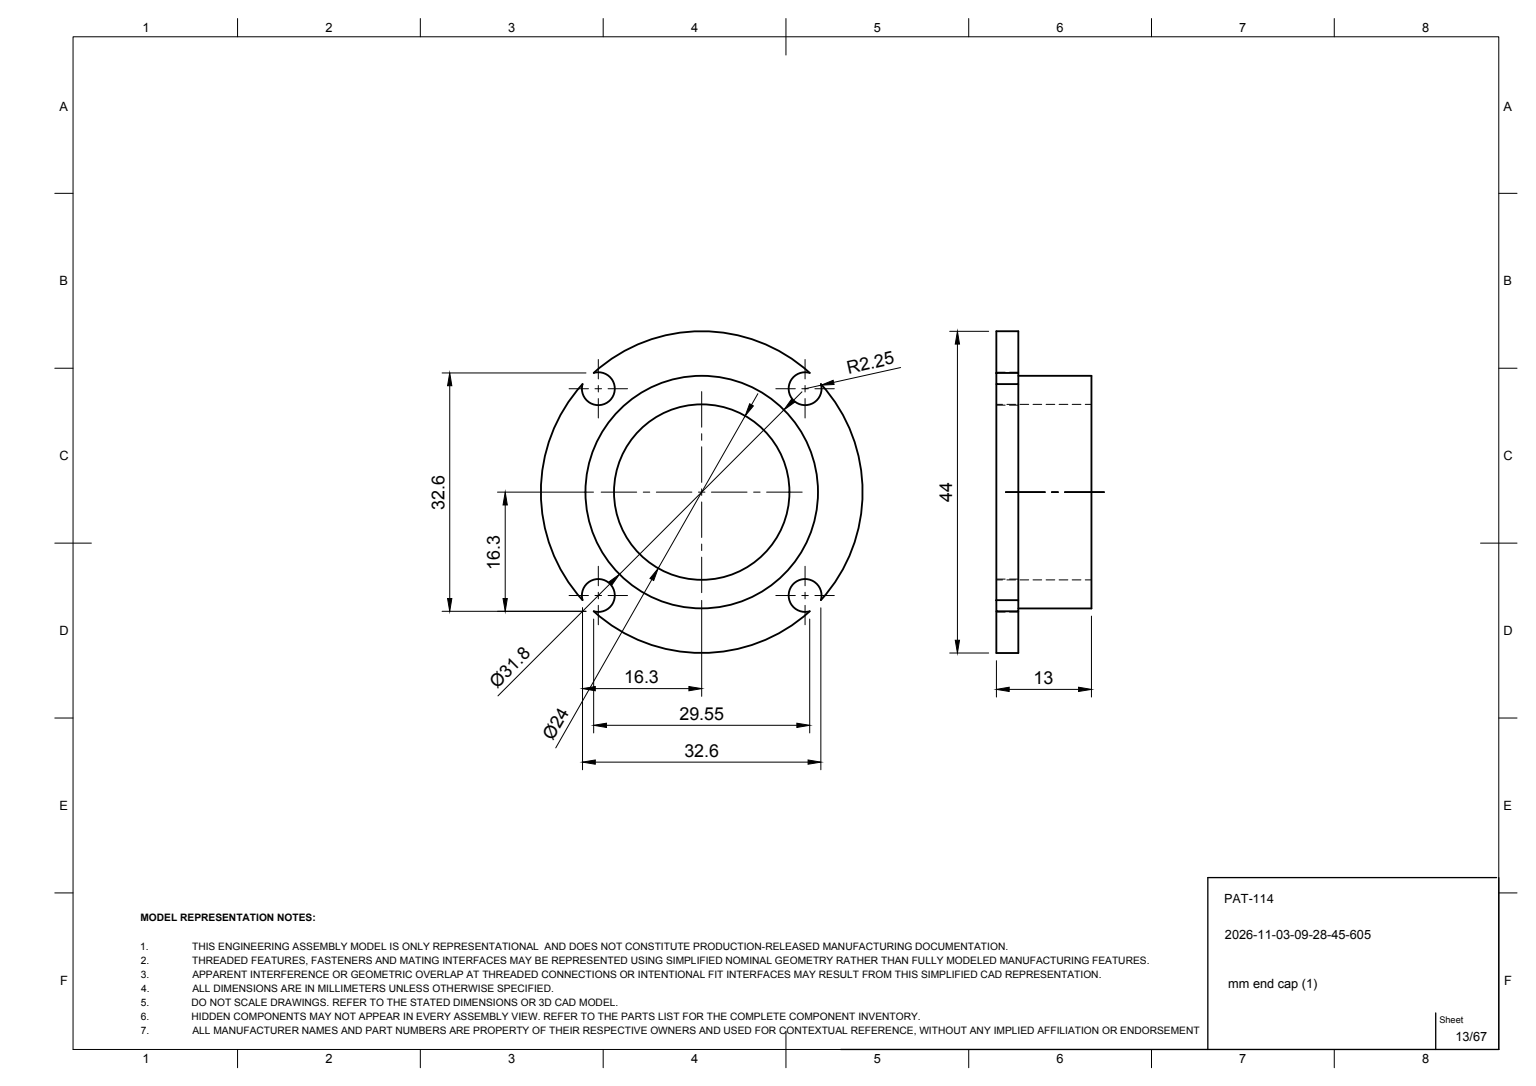
ISO-10303-21;
HEADER;
/* Generated by software containing ST-Developer
 * from STEP Tools, Inc. (www.steptools.com) 
 */

FILE_DESCRIPTION(
/* description */ ('Two-stage gear reducer in split housing'),
/* implementation_level */ '2;1');

FILE_NAME(
/* name */ 'mm end cap (1).step',
/* time_stamp */ '2026-10-28T03:22:31-07:00',
/* author */ (''),
/* organization */ (''),
/* preprocessor_version */ 'ST-DEVELOPER v20.2',
/* originating_system */ 'Autodesk Translation Framework v15.17.0.0',
/* authorisation */ '');

FILE_SCHEMA (('AUTOMOTIVE_DESIGN { 1 0 10303 214 3 1 1 }'));
ENDSEC;

DATA;
#10=MECHANICAL_DESIGN_GEOMETRIC_PRESENTATION_REPRESENTATION('',(#1242),#73366);
#1130=SHAPE_REPRESENTATION_RELATIONSHIP('SRR','None',#73617,#1186);
#1186=ADVANCED_BREP_SHAPE_REPRESENTATION('',(#1313),#73313);
#1242=STYLED_ITEM('',(#74002),#1313);
#1313=MANIFOLD_SOLID_BREP('Body1',#16130);
#1463=FACE_BOUND('',#3216,.T.);
#1464=FACE_BOUND('',#3223,.T.);
#1465=FACE_BOUND('',#3226,.T.);
#1711=PLANE('',#17238);
#1712=PLANE('',#17254);
#1713=PLANE('',#17258);
#2209=FACE_OUTER_BOUND('',#3211,.T.);
#2210=FACE_OUTER_BOUND('',#3212,.T.);
#2211=FACE_OUTER_BOUND('',#3213,.T.);
#2212=FACE_OUTER_BOUND('',#3214,.T.);
#2213=FACE_OUTER_BOUND('',#3215,.T.);
#2214=FACE_OUTER_BOUND('',#3217,.T.);
#2215=FACE_OUTER_BOUND('',#3218,.T.);
#2216=FACE_OUTER_BOUND('',#3219,.T.);
#2217=FACE_OUTER_BOUND('',#3220,.T.);
#2218=FACE_OUTER_BOUND('',#3221,.T.);
#2219=FACE_OUTER_BOUND('',#3222,.T.);
#2220=FACE_OUTER_BOUND('',#3224,.T.);
#2221=FACE_OUTER_BOUND('',#3225,.T.);
#3211=EDGE_LOOP('',(#11431,#11432,#11433,#11434));
#3212=EDGE_LOOP('',(#11435,#11436,#11437,#11438));
#3213=EDGE_LOOP('',(#11439,#11440,#11441,#11442));
#3214=EDGE_LOOP('',(#11443,#11444,#11445,#11446));
#3215=EDGE_LOOP('',(#11447,#11448,#11449,#11450,#11451,#11452,#11453,#11454));
#3216=EDGE_LOOP('',(#11455));
#3217=EDGE_LOOP('',(#11456,#11457,#11458,#11459));
#3218=EDGE_LOOP('',(#11460,#11461,#11462,#11463));
#3219=EDGE_LOOP('',(#11464,#11465,#11466,#11467));
#3220=EDGE_LOOP('',(#11468,#11469,#11470,#11471));
#3221=EDGE_LOOP('',(#11472,#11473,#11474,#11475));
#3222=EDGE_LOOP('',(#11476));
#3223=EDGE_LOOP('',(#11477));
#3224=EDGE_LOOP('',(#11478,#11479,#11480,#11481));
#3225=EDGE_LOOP('',(#11482,#11483,#11484,#11485,#11486,#11487,#11488,#11489));
#3226=EDGE_LOOP('',(#11490));
#4322=LINE('',#23765,#5346);
#4323=LINE('',#23769,#5347);
#4324=LINE('',#23774,#5348);
#4325=LINE('',#23778,#5349);
#4326=LINE('',#23783,#5350);
#4327=LINE('',#23787,#5351);
#4328=LINE('',#23792,#5352);
#4329=LINE('',#23796,#5353);
#4330=LINE('',#23815,#5354);
#4331=LINE('',#23823,#5355);
#5346=VECTOR('',#19554,1.);
#5347=VECTOR('',#19557,1.);
#5348=VECTOR('',#19562,1.);
#5349=VECTOR('',#19565,1.);
#5350=VECTOR('',#19570,1.);
#5351=VECTOR('',#19573,1.);
#5352=VECTOR('',#19578,1.);
#5353=VECTOR('',#19581,1.);
#5354=VECTOR('',#19614,1.59);
#5355=VECTOR('',#19625,1.2);
#6300=CIRCLE('',#17227,0.225);
#6301=CIRCLE('',#17228,0.225);
#6302=CIRCLE('',#17230,0.225);
#6303=CIRCLE('',#17231,0.225);
#6304=CIRCLE('',#17233,0.225);
#6305=CIRCLE('',#17234,0.225);
#6306=CIRCLE('',#17236,0.225);
#6307=CIRCLE('',#17237,0.225);
#6308=CIRCLE('',#17239,2.2);
#6309=CIRCLE('',#17240,2.2);
#6310=CIRCLE('',#17241,2.2);
#6311=CIRCLE('',#17242,2.2);
#6312=CIRCLE('',#17243,1.59);
#6313=CIRCLE('',#17245,2.2);
#6314=CIRCLE('',#17247,2.2);
#6315=CIRCLE('',#17249,2.2);
#6316=CIRCLE('',#17251,2.2);
#6317=CIRCLE('',#17253,1.59);
#6318=CIRCLE('',#17255,1.2);
#6319=CIRCLE('',#17257,1.2);
#7132=VERTEX_POINT('',#23763);
#7133=VERTEX_POINT('',#23764);
#7134=VERTEX_POINT('',#23766);
#7135=VERTEX_POINT('',#23768);
#7136=VERTEX_POINT('',#23772);
#7137=VERTEX_POINT('',#23773);
#7138=VERTEX_POINT('',#23775);
#7139=VERTEX_POINT('',#23777);
#7140=VERTEX_POINT('',#23781);
#7141=VERTEX_POINT('',#23782);
#7142=VERTEX_POINT('',#23784);
#7143=VERTEX_POINT('',#23786);
#7144=VERTEX_POINT('',#23790);
#7145=VERTEX_POINT('',#23791);
#7146=VERTEX_POINT('',#23793);
#7147=VERTEX_POINT('',#23795);
#7148=VERTEX_POINT('',#23803);
#7149=VERTEX_POINT('',#23814);
#7150=VERTEX_POINT('',#23818);
#7151=VERTEX_POINT('',#23821);
#8769=EDGE_CURVE('',#7132,#7133,#4322,.T.);
#8770=EDGE_CURVE('',#7134,#7132,#6300,.T.);
#8771=EDGE_CURVE('',#7135,#7134,#4323,.T.);
#8772=EDGE_CURVE('',#7133,#7135,#6301,.T.);
#8773=EDGE_CURVE('',#7136,#7137,#4324,.T.);
#8774=EDGE_CURVE('',#7138,#7136,#6302,.T.);
#8775=EDGE_CURVE('',#7139,#7138,#4325,.T.);
#8776=EDGE_CURVE('',#7137,#7139,#6303,.T.);
#8777=EDGE_CURVE('',#7140,#7141,#4326,.T.);
#8778=EDGE_CURVE('',#7142,#7140,#6304,.T.);
#8779=EDGE_CURVE('',#7143,#7142,#4327,.T.);
#8780=EDGE_CURVE('',#7141,#7143,#6305,.T.);
#8781=EDGE_CURVE('',#7144,#7145,#4328,.T.);
#8782=EDGE_CURVE('',#7146,#7144,#6306,.T.);
#8783=EDGE_CURVE('',#7147,#7146,#4329,.T.);
#8784=EDGE_CURVE('',#7145,#7147,#6307,.T.);
#8785=EDGE_CURVE('',#7146,#7132,#6308,.T.);
#8786=EDGE_CURVE('',#7142,#7144,#6309,.T.);
#8787=EDGE_CURVE('',#7138,#7140,#6310,.T.);
#8788=EDGE_CURVE('',#7134,#7136,#6311,.T.);
#8789=EDGE_CURVE('',#7148,#7148,#6312,.T.);
#8790=EDGE_CURVE('',#7143,#7145,#6313,.T.);
#8791=EDGE_CURVE('',#7139,#7141,#6314,.T.);
#8792=EDGE_CURVE('',#7147,#7133,#6315,.T.);
#8793=EDGE_CURVE('',#7135,#7137,#6316,.T.);
#8794=EDGE_CURVE('',#7148,#7149,#4330,.T.);
#8795=EDGE_CURVE('',#7149,#7149,#6317,.T.);
#8796=EDGE_CURVE('',#7150,#7150,#6318,.T.);
#8797=EDGE_CURVE('',#7151,#7151,#6319,.T.);
#8798=EDGE_CURVE('',#7151,#7150,#4331,.T.);
#11431=ORIENTED_EDGE('',*,*,#8769,.F.);
#11432=ORIENTED_EDGE('',*,*,#8770,.F.);
#11433=ORIENTED_EDGE('',*,*,#8771,.F.);
#11434=ORIENTED_EDGE('',*,*,#8772,.F.);
#11435=ORIENTED_EDGE('',*,*,#8773,.F.);
#11436=ORIENTED_EDGE('',*,*,#8774,.F.);
#11437=ORIENTED_EDGE('',*,*,#8775,.F.);
#11438=ORIENTED_EDGE('',*,*,#8776,.F.);
#11439=ORIENTED_EDGE('',*,*,#8777,.F.);
#11440=ORIENTED_EDGE('',*,*,#8778,.F.);
#11441=ORIENTED_EDGE('',*,*,#8779,.F.);
#11442=ORIENTED_EDGE('',*,*,#8780,.F.);
#11443=ORIENTED_EDGE('',*,*,#8781,.F.);
#11444=ORIENTED_EDGE('',*,*,#8782,.F.);
#11445=ORIENTED_EDGE('',*,*,#8783,.F.);
#11446=ORIENTED_EDGE('',*,*,#8784,.F.);
#11447=ORIENTED_EDGE('',*,*,#8770,.T.);
#11448=ORIENTED_EDGE('',*,*,#8785,.F.);
#11449=ORIENTED_EDGE('',*,*,#8782,.T.);
#11450=ORIENTED_EDGE('',*,*,#8786,.F.);
#11451=ORIENTED_EDGE('',*,*,#8778,.T.);
#11452=ORIENTED_EDGE('',*,*,#8787,.F.);
#11453=ORIENTED_EDGE('',*,*,#8774,.T.);
#11454=ORIENTED_EDGE('',*,*,#8788,.F.);
#11455=ORIENTED_EDGE('',*,*,#8789,.T.);
#11456=ORIENTED_EDGE('',*,*,#8779,.T.);
#11457=ORIENTED_EDGE('',*,*,#8786,.T.);
#11458=ORIENTED_EDGE('',*,*,#8781,.T.);
#11459=ORIENTED_EDGE('',*,*,#8790,.F.);
#11460=ORIENTED_EDGE('',*,*,#8775,.T.);
#11461=ORIENTED_EDGE('',*,*,#8787,.T.);
#11462=ORIENTED_EDGE('',*,*,#8777,.T.);
#11463=ORIENTED_EDGE('',*,*,#8791,.F.);
#11464=ORIENTED_EDGE('',*,*,#8769,.T.);
#11465=ORIENTED_EDGE('',*,*,#8792,.F.);
#11466=ORIENTED_EDGE('',*,*,#8783,.T.);
#11467=ORIENTED_EDGE('',*,*,#8785,.T.);
#11468=ORIENTED_EDGE('',*,*,#8771,.T.);
#11469=ORIENTED_EDGE('',*,*,#8788,.T.);
#11470=ORIENTED_EDGE('',*,*,#8773,.T.);
#11471=ORIENTED_EDGE('',*,*,#8793,.F.);
#11472=ORIENTED_EDGE('',*,*,#8789,.F.);
#11473=ORIENTED_EDGE('',*,*,#8794,.T.);
#11474=ORIENTED_EDGE('',*,*,#8795,.T.);
#11475=ORIENTED_EDGE('',*,*,#8794,.F.);
#11476=ORIENTED_EDGE('',*,*,#8795,.F.);
#11477=ORIENTED_EDGE('',*,*,#8796,.F.);
#11478=ORIENTED_EDGE('',*,*,#8797,.F.);
#11479=ORIENTED_EDGE('',*,*,#8798,.T.);
#11480=ORIENTED_EDGE('',*,*,#8796,.T.);
#11481=ORIENTED_EDGE('',*,*,#8798,.F.);
#11482=ORIENTED_EDGE('',*,*,#8772,.T.);
#11483=ORIENTED_EDGE('',*,*,#8793,.T.);
#11484=ORIENTED_EDGE('',*,*,#8776,.T.);
#11485=ORIENTED_EDGE('',*,*,#8791,.T.);
#11486=ORIENTED_EDGE('',*,*,#8780,.T.);
#11487=ORIENTED_EDGE('',*,*,#8790,.T.);
#11488=ORIENTED_EDGE('',*,*,#8784,.T.);
#11489=ORIENTED_EDGE('',*,*,#8792,.T.);
#11490=ORIENTED_EDGE('',*,*,#8797,.T.);
#15005=CYLINDRICAL_SURFACE('',#17226,0.225);
#15006=CYLINDRICAL_SURFACE('',#17229,0.225);
#15007=CYLINDRICAL_SURFACE('',#17232,0.225);
#15008=CYLINDRICAL_SURFACE('',#17235,0.225);
#15009=CYLINDRICAL_SURFACE('',#17244,2.2);
#15010=CYLINDRICAL_SURFACE('',#17246,2.2);
#15011=CYLINDRICAL_SURFACE('',#17248,2.2);
#15012=CYLINDRICAL_SURFACE('',#17250,2.2);
#15013=CYLINDRICAL_SURFACE('',#17252,1.59);
#15014=CYLINDRICAL_SURFACE('',#17256,1.2);
#15416=ADVANCED_FACE('',(#2209),#15005,.F.);
#15417=ADVANCED_FACE('',(#2210),#15006,.F.);
#15418=ADVANCED_FACE('',(#2211),#15007,.F.);
#15419=ADVANCED_FACE('',(#2212),#15008,.F.);
#15420=ADVANCED_FACE('',(#2213,#1463),#1711,.F.);
#15421=ADVANCED_FACE('',(#2214),#15009,.T.);
#15422=ADVANCED_FACE('',(#2215),#15010,.T.);
#15423=ADVANCED_FACE('',(#2216),#15011,.T.);
#15424=ADVANCED_FACE('',(#2217),#15012,.T.);
#15425=ADVANCED_FACE('',(#2218),#15013,.T.);
#15426=ADVANCED_FACE('',(#2219,#1464),#1712,.F.);
#15427=ADVANCED_FACE('',(#2220),#15014,.F.);
#15428=ADVANCED_FACE('',(#2221,#1465),#1713,.T.);
#16130=CLOSED_SHELL('',(#15416,#15417,#15418,#15419,#15420,#15421,#15422,
#15423,#15424,#15425,#15426,#15427,#15428));
#17225=AXIS2_PLACEMENT_3D('',#23761,#19550,#19551);
#17226=AXIS2_PLACEMENT_3D('',#23762,#19552,#19553);
#17227=AXIS2_PLACEMENT_3D('',#23767,#19555,#19556);
#17228=AXIS2_PLACEMENT_3D('',#23770,#19558,#19559);
#17229=AXIS2_PLACEMENT_3D('',#23771,#19560,#19561);
#17230=AXIS2_PLACEMENT_3D('',#23776,#19563,#19564);
#17231=AXIS2_PLACEMENT_3D('',#23779,#19566,#19567);
#17232=AXIS2_PLACEMENT_3D('',#23780,#19568,#19569);
#17233=AXIS2_PLACEMENT_3D('',#23785,#19571,#19572);
#17234=AXIS2_PLACEMENT_3D('',#23788,#19574,#19575);
#17235=AXIS2_PLACEMENT_3D('',#23789,#19576,#19577);
#17236=AXIS2_PLACEMENT_3D('',#23794,#19579,#19580);
#17237=AXIS2_PLACEMENT_3D('',#23797,#19582,#19583);
#17238=AXIS2_PLACEMENT_3D('',#23798,#19584,#19585);
#17239=AXIS2_PLACEMENT_3D('',#23799,#19586,#19587);
#17240=AXIS2_PLACEMENT_3D('',#23800,#19588,#19589);
#17241=AXIS2_PLACEMENT_3D('',#23801,#19590,#19591);
#17242=AXIS2_PLACEMENT_3D('',#23802,#19592,#19593);
#17243=AXIS2_PLACEMENT_3D('',#23804,#19594,#19595);
#17244=AXIS2_PLACEMENT_3D('',#23805,#19596,#19597);
#17245=AXIS2_PLACEMENT_3D('',#23806,#19598,#19599);
#17246=AXIS2_PLACEMENT_3D('',#23807,#19600,#19601);
#17247=AXIS2_PLACEMENT_3D('',#23808,#19602,#19603);
#17248=AXIS2_PLACEMENT_3D('',#23809,#19604,#19605);
#17249=AXIS2_PLACEMENT_3D('',#23810,#19606,#19607);
#17250=AXIS2_PLACEMENT_3D('',#23811,#19608,#19609);
#17251=AXIS2_PLACEMENT_3D('',#23812,#19610,#19611);
#17252=AXIS2_PLACEMENT_3D('',#23813,#19612,#19613);
#17253=AXIS2_PLACEMENT_3D('',#23816,#19615,#19616);
#17254=AXIS2_PLACEMENT_3D('',#23817,#19617,#19618);
#17255=AXIS2_PLACEMENT_3D('',#23819,#19619,#19620);
#17256=AXIS2_PLACEMENT_3D('',#23820,#19621,#19622);
#17257=AXIS2_PLACEMENT_3D('',#23822,#19623,#19624);
#17258=AXIS2_PLACEMENT_3D('',#23824,#19626,#19627);
#19550=DIRECTION('axis',(0.,0.,1.));
#19551=DIRECTION('refdir',(1.,0.,0.));
#19552=DIRECTION('center_axis',(0.,1.,0.));
#19553=DIRECTION('ref_axis',(0.707106781186543,0.,0.707106781186552));
#19554=DIRECTION('',(0.,1.,0.));
#19555=DIRECTION('center_axis',(0.,1.,0.));
#19556=DIRECTION('ref_axis',(1.,0.,0.));
#19557=DIRECTION('',(0.,-1.,0.));
#19558=DIRECTION('center_axis',(0.,-1.,0.));
#19559=DIRECTION('ref_axis',(1.,0.,0.));
#19560=DIRECTION('center_axis',(0.,1.,0.));
#19561=DIRECTION('ref_axis',(0.707106781186542,0.,-0.707106781186553));
#19562=DIRECTION('',(0.,1.,0.));
#19563=DIRECTION('center_axis',(0.,1.,0.));
#19564=DIRECTION('ref_axis',(1.,0.,0.));
#19565=DIRECTION('',(0.,-1.,0.));
#19566=DIRECTION('center_axis',(0.,-1.,0.));
#19567=DIRECTION('ref_axis',(1.,0.,0.));
#19568=DIRECTION('center_axis',(0.,1.,0.));
#19569=DIRECTION('ref_axis',(-0.707106781186542,0.,-0.707106781186553));
#19570=DIRECTION('',(0.,1.,0.));
#19571=DIRECTION('center_axis',(0.,1.,0.));
#19572=DIRECTION('ref_axis',(1.,0.,0.));
#19573=DIRECTION('',(0.,-1.,0.));
#19574=DIRECTION('center_axis',(0.,-1.,0.));
#19575=DIRECTION('ref_axis',(1.,0.,0.));
#19576=DIRECTION('center_axis',(0.,1.,0.));
#19577=DIRECTION('ref_axis',(-0.707106781186549,0.,0.707106781186546));
#19578=DIRECTION('',(0.,1.,0.));
#19579=DIRECTION('center_axis',(0.,1.,0.));
#19580=DIRECTION('ref_axis',(1.,0.,0.));
#19581=DIRECTION('',(0.,-1.,0.));
#19582=DIRECTION('center_axis',(0.,-1.,0.));
#19583=DIRECTION('ref_axis',(1.,0.,0.));
#19584=DIRECTION('center_axis',(0.,1.,0.));
#19585=DIRECTION('ref_axis',(1.,0.,0.));
#19586=DIRECTION('center_axis',(0.,1.,0.));
#19587=DIRECTION('ref_axis',(1.,0.,0.));
#19588=DIRECTION('center_axis',(0.,1.,0.));
#19589=DIRECTION('ref_axis',(1.,0.,0.));
#19590=DIRECTION('center_axis',(0.,1.,0.));
#19591=DIRECTION('ref_axis',(1.,0.,0.));
#19592=DIRECTION('center_axis',(0.,1.,0.));
#19593=DIRECTION('ref_axis',(1.,0.,0.));
#19594=DIRECTION('center_axis',(0.,1.,0.));
#19595=DIRECTION('ref_axis',(1.,0.,0.));
#19596=DIRECTION('center_axis',(0.,1.,0.));
#19597=DIRECTION('ref_axis',(1.,0.,0.));
#19598=DIRECTION('center_axis',(0.,1.,0.));
#19599=DIRECTION('ref_axis',(1.,0.,0.));
#19600=DIRECTION('center_axis',(0.,1.,0.));
#19601=DIRECTION('ref_axis',(1.,0.,0.));
#19602=DIRECTION('center_axis',(0.,1.,0.));
#19603=DIRECTION('ref_axis',(1.,0.,0.));
#19604=DIRECTION('center_axis',(0.,1.,0.));
#19605=DIRECTION('ref_axis',(1.,0.,0.));
#19606=DIRECTION('center_axis',(0.,1.,0.));
#19607=DIRECTION('ref_axis',(1.,0.,0.));
#19608=DIRECTION('center_axis',(0.,1.,0.));
#19609=DIRECTION('ref_axis',(-1.,0.,3.21624529935327E-16));
#19610=DIRECTION('center_axis',(0.,1.,0.));
#19611=DIRECTION('ref_axis',(1.,0.,0.));
#19612=DIRECTION('center_axis',(0.,1.,0.));
#19613=DIRECTION('ref_axis',(1.,0.,0.));
#19614=DIRECTION('',(0.,-1.,0.));
#19615=DIRECTION('center_axis',(0.,1.,0.));
#19616=DIRECTION('ref_axis',(1.,0.,0.));
#19617=DIRECTION('center_axis',(0.,1.,0.));
#19618=DIRECTION('ref_axis',(1.,0.,0.));
#19619=DIRECTION('center_axis',(0.,-1.,0.));
#19620=DIRECTION('ref_axis',(1.,0.,0.));
#19621=DIRECTION('center_axis',(0.,1.,0.));
#19622=DIRECTION('ref_axis',(1.,0.,0.));
#19623=DIRECTION('center_axis',(0.,-1.,0.));
#19624=DIRECTION('ref_axis',(1.,0.,0.));
#19625=DIRECTION('',(0.,-1.,0.));
#19626=DIRECTION('center_axis',(0.,1.,0.));
#19627=DIRECTION('ref_axis',(1.,0.,0.));
#23761=CARTESIAN_POINT('',(0.,0.,0.));
#23762=CARTESIAN_POINT('Origin',(-1.4142135623731,7.4,8.5857864376269));
#23763=CARTESIAN_POINT('',(-1.47733531993816,7.5,8.3698219874924));
#23764=CARTESIAN_POINT('',(-1.47733531993816,7.8,8.3698219874924));
#23765=CARTESIAN_POINT('',(-1.47733531993816,7.4,8.3698219874924));
#23766=CARTESIAN_POINT('',(-1.6301780125076,7.5,8.52266468006184));
#23767=CARTESIAN_POINT('Origin',(-1.4142135623731,7.5,8.5857864376269));
#23768=CARTESIAN_POINT('',(-1.6301780125076,7.8,8.52266468006184));
#23769=CARTESIAN_POINT('',(-1.6301780125076,7.4,8.52266468006184));
#23770=CARTESIAN_POINT('Origin',(-1.4142135623731,7.8,8.5857864376269));
#23771=CARTESIAN_POINT('Origin',(-1.41421356237309,7.4,11.4142135623731));
#23772=CARTESIAN_POINT('',(-1.6301780125076,7.5,11.4773353199382));
#23773=CARTESIAN_POINT('',(-1.6301780125076,7.8,11.4773353199382));
#23774=CARTESIAN_POINT('',(-1.6301780125076,7.4,11.4773353199382));
#23775=CARTESIAN_POINT('',(-1.47733531993816,7.5,11.6301780125076));
#23776=CARTESIAN_POINT('Origin',(-1.41421356237309,7.5,11.4142135623731));
#23777=CARTESIAN_POINT('',(-1.47733531993816,7.8,11.6301780125076));
#23778=CARTESIAN_POINT('',(-1.47733531993816,7.4,11.6301780125076));
#23779=CARTESIAN_POINT('Origin',(-1.41421356237309,7.8,11.4142135623731));
#23780=CARTESIAN_POINT('Origin',(1.4142135623731,7.4,11.4142135623731));
#23781=CARTESIAN_POINT('',(1.47733531993816,7.5,11.6301780125076));
#23782=CARTESIAN_POINT('',(1.47733531993816,7.8,11.6301780125076));
#23783=CARTESIAN_POINT('',(1.47733531993816,7.4,11.6301780125076));
#23784=CARTESIAN_POINT('',(1.6301780125076,7.5,11.4773353199382));
#23785=CARTESIAN_POINT('Origin',(1.4142135623731,7.5,11.4142135623731));
#23786=CARTESIAN_POINT('',(1.6301780125076,7.8,11.4773353199382));
#23787=CARTESIAN_POINT('',(1.6301780125076,7.4,11.4773353199382));
#23788=CARTESIAN_POINT('Origin',(1.4142135623731,7.8,11.4142135623731));
#23789=CARTESIAN_POINT('Origin',(1.41421356237309,7.4,8.5857864376269));
#23790=CARTESIAN_POINT('',(1.6301780125076,7.5,8.52266468006184));
#23791=CARTESIAN_POINT('',(1.6301780125076,7.8,8.52266468006184));
#23792=CARTESIAN_POINT('',(1.6301780125076,7.4,8.52266468006184));
#23793=CARTESIAN_POINT('',(1.47733531993816,7.5,8.3698219874924));
#23794=CARTESIAN_POINT('Origin',(1.41421356237309,7.5,8.5857864376269));
#23795=CARTESIAN_POINT('',(1.47733531993816,7.8,8.3698219874924));
#23796=CARTESIAN_POINT('',(1.47733531993816,7.4,8.3698219874924));
#23797=CARTESIAN_POINT('Origin',(1.41421356237309,7.8,8.5857864376269));
#23798=CARTESIAN_POINT('Origin',(0.,7.5,10.));
#23799=CARTESIAN_POINT('Origin',(0.,7.5,10.));
#23800=CARTESIAN_POINT('Origin',(0.,7.5,10.));
#23801=CARTESIAN_POINT('Origin',(0.,7.5,10.));
#23802=CARTESIAN_POINT('Origin',(0.,7.5,10.));
#23803=CARTESIAN_POINT('',(-1.59,7.5,10.));
#23804=CARTESIAN_POINT('Origin',(0.,7.5,10.));
#23805=CARTESIAN_POINT('Origin',(0.,7.5,10.));
#23806=CARTESIAN_POINT('Origin',(0.,7.8,10.));
#23807=CARTESIAN_POINT('Origin',(0.,7.5,10.));
#23808=CARTESIAN_POINT('Origin',(0.,7.8,10.));
#23809=CARTESIAN_POINT('Origin',(0.,7.5,10.));
#23810=CARTESIAN_POINT('Origin',(0.,7.8,10.));
#23811=CARTESIAN_POINT('Origin',(0.,7.5,10.));
#23812=CARTESIAN_POINT('Origin',(0.,7.8,10.));
#23813=CARTESIAN_POINT('Origin',(0.,6.5,10.));
#23814=CARTESIAN_POINT('',(-1.59,6.5,10.));
#23815=CARTESIAN_POINT('',(-1.59,6.5,10.));
#23816=CARTESIAN_POINT('Origin',(0.,6.5,10.));
#23817=CARTESIAN_POINT('Origin',(0.,6.5,10.));
#23818=CARTESIAN_POINT('',(-1.2,6.5,10.));
#23819=CARTESIAN_POINT('Origin',(0.,6.5,10.));
#23820=CARTESIAN_POINT('Origin',(0.,7.5,10.));
#23821=CARTESIAN_POINT('',(-1.2,7.8,10.));
#23822=CARTESIAN_POINT('Origin',(0.,7.8,10.));
#23823=CARTESIAN_POINT('',(-1.2,7.5,10.));
#23824=CARTESIAN_POINT('Origin',(0.,7.8,10.));
#73249=UNCERTAINTY_MEASURE_WITH_UNIT(LENGTH_MEASURE(0.001),#73367,
'DISTANCE_ACCURACY_VALUE',
'Maximum model space distance between geometric entities at asserted c
onnectivities');
#73302=UNCERTAINTY_MEASURE_WITH_UNIT(LENGTH_MEASURE(0.001),#73367,
'DISTANCE_ACCURACY_VALUE',
'Maximum model space distance between geometric entities at asserted c
onnectivities');
#73313=(
GEOMETRIC_REPRESENTATION_CONTEXT(3)
GLOBAL_UNCERTAINTY_ASSIGNED_CONTEXT((#73249))
GLOBAL_UNIT_ASSIGNED_CONTEXT((#73367,#73369,#73370))
REPRESENTATION_CONTEXT('','3D')
);
#73366=(
GEOMETRIC_REPRESENTATION_CONTEXT(3)
GLOBAL_UNCERTAINTY_ASSIGNED_CONTEXT((#73302))
GLOBAL_UNIT_ASSIGNED_CONTEXT((#73367,#73369,#73370))
REPRESENTATION_CONTEXT('','3D')
);
#73367=(
LENGTH_UNIT()
NAMED_UNIT(*)
SI_UNIT(.CENTI.,.METRE.)
);
#73369=(
NAMED_UNIT(*)
PLANE_ANGLE_UNIT()
SI_UNIT($,.RADIAN.)
);
#73370=(
NAMED_UNIT(*)
SI_UNIT($,.STERADIAN.)
SOLID_ANGLE_UNIT()
);
#73381=SHAPE_DEFINITION_REPRESENTATION(#73444,#73617);
#73444=PRODUCT_DEFINITION_SHAPE('',$,#73681);
#73617=SHAPE_REPRESENTATION('',(#17225),#73313);
#73670=PRODUCT_DEFINITION_CONTEXT('part definition',#73861,'design');
#73681=PRODUCT_DEFINITION('mm end cap (1)','mm end cap (1)',#73744,#73670);
#73744=PRODUCT_DEFINITION_FORMATION('',$,#73873);
#73861=APPLICATION_CONTEXT(
'Core Data for Automotive Mechanical Design Process');
#73862=PRODUCT_CONTEXT('part definition',#73861,'mechanical');
#73873=PRODUCT('mm end cap (1)','mm end cap (1)','mm end cap (1)',(#73862));
#73996=COLOUR_RGB('Off White',0.89,0.88,0.83);
#73997=FILL_AREA_STYLE_COLOUR('',#73996);
#73998=FILL_AREA_STYLE('',(#73997));
#73999=SURFACE_STYLE_FILL_AREA(#73998);
#74000=SURFACE_SIDE_STYLE('',(#73999));
#74001=SURFACE_STYLE_USAGE(.BOTH.,#74000);
#74002=PRESENTATION_STYLE_ASSIGNMENT((#74001));
ENDSEC;
END-ISO-10303-21;
